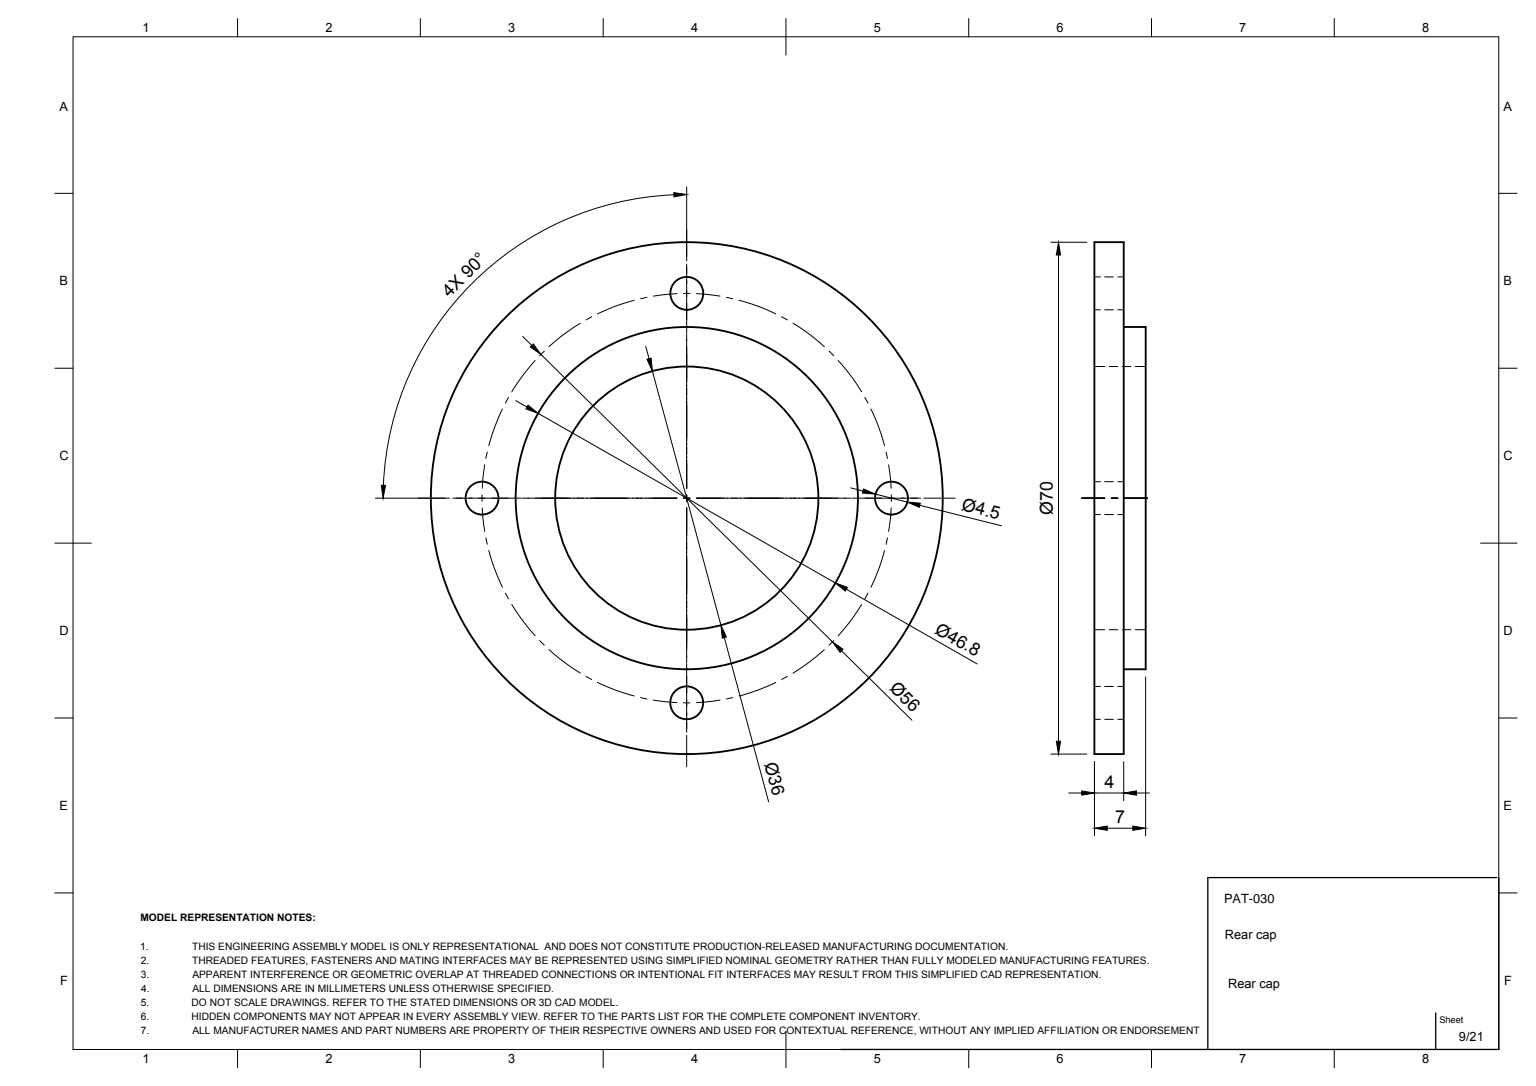
ISO-10303-21;
HEADER;
/* Generated by software containing ST-Developer
 * from STEP Tools, Inc. (www.steptools.com) 
 */

FILE_DESCRIPTION(
/* description */ ('Double-bearing flanged cartridge'),
/* implementation_level */ '2;1');

FILE_NAME(
/* name */ 'Rear cap.step',
/* time_stamp */ '2026-10-28T03:26:40-07:00',
/* author */ (''),
/* organization */ (''),
/* preprocessor_version */ 'ST-DEVELOPER v20.2',
/* originating_system */ 'Autodesk Translation Framework v15.17.0.0',
/* authorisation */ '');

FILE_SCHEMA (('AUTOMOTIVE_DESIGN { 1 0 10303 214 3 1 1 }'));
ENDSEC;

DATA;
#10=MECHANICAL_DESIGN_GEOMETRIC_PRESENTATION_REPRESENTATION('',(#207),#5535);
#171=SHAPE_REPRESENTATION_RELATIONSHIP('SRR','None',#5613,#185);
#185=ADVANCED_BREP_SHAPE_REPRESENTATION('',(#229),#5529);
#207=STYLED_ITEM('',(#5757),#229);
#229=MANIFOLD_SOLID_BREP('Body1',#2341);
#278=FACE_BOUND('',#660,.T.);
#279=FACE_BOUND('',#664,.T.);
#280=FACE_BOUND('',#665,.T.);
#281=FACE_BOUND('',#666,.T.);
#282=FACE_BOUND('',#667,.T.);
#283=FACE_BOUND('',#668,.T.);
#284=FACE_BOUND('',#670,.T.);
#285=FACE_BOUND('',#671,.T.);
#286=FACE_BOUND('',#672,.T.);
#287=FACE_BOUND('',#673,.T.);
#288=FACE_BOUND('',#674,.T.);
#337=PLANE('',#2762);
#338=PLANE('',#2769);
#339=PLANE('',#2770);
#460=FACE_OUTER_BOUND('',#654,.T.);
#461=FACE_OUTER_BOUND('',#655,.T.);
#462=FACE_OUTER_BOUND('',#656,.T.);
#463=FACE_OUTER_BOUND('',#657,.T.);
#464=FACE_OUTER_BOUND('',#658,.T.);
#465=FACE_OUTER_BOUND('',#659,.T.);
#466=FACE_OUTER_BOUND('',#661,.T.);
#467=FACE_OUTER_BOUND('',#662,.T.);
#468=FACE_OUTER_BOUND('',#663,.T.);
#469=FACE_OUTER_BOUND('',#669,.T.);
#654=EDGE_LOOP('',(#1930,#1931,#1932,#1933));
#655=EDGE_LOOP('',(#1934,#1935,#1936,#1937));
#656=EDGE_LOOP('',(#1938,#1939,#1940,#1941));
#657=EDGE_LOOP('',(#1942,#1943,#1944,#1945));
#658=EDGE_LOOP('',(#1946,#1947,#1948,#1949));
#659=EDGE_LOOP('',(#1950));
#660=EDGE_LOOP('',(#1951));
#661=EDGE_LOOP('',(#1952,#1953,#1954,#1955));
#662=EDGE_LOOP('',(#1956,#1957,#1958,#1959));
#663=EDGE_LOOP('',(#1960));
#664=EDGE_LOOP('',(#1961));
#665=EDGE_LOOP('',(#1962));
#666=EDGE_LOOP('',(#1963));
#667=EDGE_LOOP('',(#1964));
#668=EDGE_LOOP('',(#1965));
#669=EDGE_LOOP('',(#1966));
#670=EDGE_LOOP('',(#1967));
#671=EDGE_LOOP('',(#1968));
#672=EDGE_LOOP('',(#1969));
#673=EDGE_LOOP('',(#1970));
#674=EDGE_LOOP('',(#1971));
#770=LINE('',#4468,#856);
#771=LINE('',#4474,#857);
#772=LINE('',#4480,#858);
#773=LINE('',#4486,#859);
#774=LINE('',#4492,#860);
#775=LINE('',#4500,#861);
#776=LINE('',#4505,#862);
#856=VECTOR('',#3405,0.225);
#857=VECTOR('',#3412,0.225);
#858=VECTOR('',#3419,0.225);
#859=VECTOR('',#3426,0.225);
#860=VECTOR('',#3433,2.34);
#861=VECTOR('',#3444,1.8);
#862=VECTOR('',#3449,3.5);
#1026=CIRCLE('',#2748,0.225);
#1027=CIRCLE('',#2749,0.225);
#1028=CIRCLE('',#2751,0.225);
#1029=CIRCLE('',#2752,0.225);
#1030=CIRCLE('',#2754,0.225);
#1031=CIRCLE('',#2755,0.225);
#1032=CIRCLE('',#2757,0.225);
#1033=CIRCLE('',#2758,0.225);
#1034=CIRCLE('',#2760,2.34);
#1035=CIRCLE('',#2761,2.34);
#1036=CIRCLE('',#2763,1.8);
#1037=CIRCLE('',#2765,1.8);
#1038=CIRCLE('',#2767,3.5);
#1039=CIRCLE('',#2768,3.5);
#1208=VERTEX_POINT('',#4465);
#1209=VERTEX_POINT('',#4467);
#1210=VERTEX_POINT('',#4471);
#1211=VERTEX_POINT('',#4473);
#1212=VERTEX_POINT('',#4477);
#1213=VERTEX_POINT('',#4479);
#1214=VERTEX_POINT('',#4483);
#1215=VERTEX_POINT('',#4485);
#1216=VERTEX_POINT('',#4489);
#1217=VERTEX_POINT('',#4491);
#1218=VERTEX_POINT('',#4495);
#1219=VERTEX_POINT('',#4498);
#1220=VERTEX_POINT('',#4502);
#1221=VERTEX_POINT('',#4504);
#1458=EDGE_CURVE('',#1208,#1208,#1026,.T.);
#1459=EDGE_CURVE('',#1208,#1209,#770,.T.);
#1460=EDGE_CURVE('',#1209,#1209,#1027,.T.);
#1461=EDGE_CURVE('',#1210,#1210,#1028,.T.);
#1462=EDGE_CURVE('',#1210,#1211,#771,.T.);
#1463=EDGE_CURVE('',#1211,#1211,#1029,.T.);
#1464=EDGE_CURVE('',#1212,#1212,#1030,.T.);
#1465=EDGE_CURVE('',#1212,#1213,#772,.T.);
#1466=EDGE_CURVE('',#1213,#1213,#1031,.T.);
#1467=EDGE_CURVE('',#1214,#1214,#1032,.T.);
#1468=EDGE_CURVE('',#1214,#1215,#773,.T.);
#1469=EDGE_CURVE('',#1215,#1215,#1033,.T.);
#1470=EDGE_CURVE('',#1216,#1216,#1034,.T.);
#1471=EDGE_CURVE('',#1216,#1217,#774,.T.);
#1472=EDGE_CURVE('',#1217,#1217,#1035,.T.);
#1473=EDGE_CURVE('',#1218,#1218,#1036,.T.);
#1474=EDGE_CURVE('',#1219,#1219,#1037,.T.);
#1475=EDGE_CURVE('',#1219,#1218,#775,.T.);
#1476=EDGE_CURVE('',#1220,#1220,#1038,.T.);
#1477=EDGE_CURVE('',#1220,#1221,#776,.T.);
#1478=EDGE_CURVE('',#1221,#1221,#1039,.T.);
#1930=ORIENTED_EDGE('',*,*,#1458,.F.);
#1931=ORIENTED_EDGE('',*,*,#1459,.T.);
#1932=ORIENTED_EDGE('',*,*,#1460,.F.);
#1933=ORIENTED_EDGE('',*,*,#1459,.F.);
#1934=ORIENTED_EDGE('',*,*,#1461,.F.);
#1935=ORIENTED_EDGE('',*,*,#1462,.T.);
#1936=ORIENTED_EDGE('',*,*,#1463,.F.);
#1937=ORIENTED_EDGE('',*,*,#1462,.F.);
#1938=ORIENTED_EDGE('',*,*,#1464,.F.);
#1939=ORIENTED_EDGE('',*,*,#1465,.T.);
#1940=ORIENTED_EDGE('',*,*,#1466,.F.);
#1941=ORIENTED_EDGE('',*,*,#1465,.F.);
#1942=ORIENTED_EDGE('',*,*,#1467,.F.);
#1943=ORIENTED_EDGE('',*,*,#1468,.T.);
#1944=ORIENTED_EDGE('',*,*,#1469,.F.);
#1945=ORIENTED_EDGE('',*,*,#1468,.F.);
#1946=ORIENTED_EDGE('',*,*,#1470,.F.);
#1947=ORIENTED_EDGE('',*,*,#1471,.T.);
#1948=ORIENTED_EDGE('',*,*,#1472,.T.);
#1949=ORIENTED_EDGE('',*,*,#1471,.F.);
#1950=ORIENTED_EDGE('',*,*,#1472,.F.);
#1951=ORIENTED_EDGE('',*,*,#1473,.F.);
#1952=ORIENTED_EDGE('',*,*,#1474,.F.);
#1953=ORIENTED_EDGE('',*,*,#1475,.T.);
#1954=ORIENTED_EDGE('',*,*,#1473,.T.);
#1955=ORIENTED_EDGE('',*,*,#1475,.F.);
#1956=ORIENTED_EDGE('',*,*,#1476,.F.);
#1957=ORIENTED_EDGE('',*,*,#1477,.T.);
#1958=ORIENTED_EDGE('',*,*,#1478,.T.);
#1959=ORIENTED_EDGE('',*,*,#1477,.F.);
#1960=ORIENTED_EDGE('',*,*,#1476,.T.);
#1961=ORIENTED_EDGE('',*,*,#1474,.T.);
#1962=ORIENTED_EDGE('',*,*,#1469,.T.);
#1963=ORIENTED_EDGE('',*,*,#1466,.T.);
#1964=ORIENTED_EDGE('',*,*,#1463,.T.);
#1965=ORIENTED_EDGE('',*,*,#1460,.T.);
#1966=ORIENTED_EDGE('',*,*,#1478,.F.);
#1967=ORIENTED_EDGE('',*,*,#1470,.T.);
#1968=ORIENTED_EDGE('',*,*,#1467,.T.);
#1969=ORIENTED_EDGE('',*,*,#1464,.T.);
#1970=ORIENTED_EDGE('',*,*,#1461,.T.);
#1971=ORIENTED_EDGE('',*,*,#1458,.T.);
#2154=CYLINDRICAL_SURFACE('',#2747,0.225);
#2155=CYLINDRICAL_SURFACE('',#2750,0.225);
#2156=CYLINDRICAL_SURFACE('',#2753,0.225);
#2157=CYLINDRICAL_SURFACE('',#2756,0.225);
#2158=CYLINDRICAL_SURFACE('',#2759,2.34);
#2159=CYLINDRICAL_SURFACE('',#2764,1.8);
#2160=CYLINDRICAL_SURFACE('',#2766,3.5);
#2274=ADVANCED_FACE('',(#460),#2154,.F.);
#2275=ADVANCED_FACE('',(#461),#2155,.F.);
#2276=ADVANCED_FACE('',(#462),#2156,.F.);
#2277=ADVANCED_FACE('',(#463),#2157,.F.);
#2278=ADVANCED_FACE('',(#464),#2158,.T.);
#2279=ADVANCED_FACE('',(#465,#278),#337,.F.);
#2280=ADVANCED_FACE('',(#466),#2159,.F.);
#2281=ADVANCED_FACE('',(#467),#2160,.T.);
#2282=ADVANCED_FACE('',(#468,#279,#280,#281,#282,#283),#338,.T.);
#2283=ADVANCED_FACE('',(#469,#284,#285,#286,#287,#288),#339,.F.);
#2341=CLOSED_SHELL('',(#2274,#2275,#2276,#2277,#2278,#2279,#2280,#2281,
#2282,#2283));
#2746=AXIS2_PLACEMENT_3D('',#4463,#3399,#3400);
#2747=AXIS2_PLACEMENT_3D('',#4464,#3401,#3402);
#2748=AXIS2_PLACEMENT_3D('',#4466,#3403,#3404);
#2749=AXIS2_PLACEMENT_3D('',#4469,#3406,#3407);
#2750=AXIS2_PLACEMENT_3D('',#4470,#3408,#3409);
#2751=AXIS2_PLACEMENT_3D('',#4472,#3410,#3411);
#2752=AXIS2_PLACEMENT_3D('',#4475,#3413,#3414);
#2753=AXIS2_PLACEMENT_3D('',#4476,#3415,#3416);
#2754=AXIS2_PLACEMENT_3D('',#4478,#3417,#3418);
#2755=AXIS2_PLACEMENT_3D('',#4481,#3420,#3421);
#2756=AXIS2_PLACEMENT_3D('',#4482,#3422,#3423);
#2757=AXIS2_PLACEMENT_3D('',#4484,#3424,#3425);
#2758=AXIS2_PLACEMENT_3D('',#4487,#3427,#3428);
#2759=AXIS2_PLACEMENT_3D('',#4488,#3429,#3430);
#2760=AXIS2_PLACEMENT_3D('',#4490,#3431,#3432);
#2761=AXIS2_PLACEMENT_3D('',#4493,#3434,#3435);
#2762=AXIS2_PLACEMENT_3D('',#4494,#3436,#3437);
#2763=AXIS2_PLACEMENT_3D('',#4496,#3438,#3439);
#2764=AXIS2_PLACEMENT_3D('',#4497,#3440,#3441);
#2765=AXIS2_PLACEMENT_3D('',#4499,#3442,#3443);
#2766=AXIS2_PLACEMENT_3D('',#4501,#3445,#3446);
#2767=AXIS2_PLACEMENT_3D('',#4503,#3447,#3448);
#2768=AXIS2_PLACEMENT_3D('',#4506,#3450,#3451);
#2769=AXIS2_PLACEMENT_3D('',#4507,#3452,#3453);
#2770=AXIS2_PLACEMENT_3D('',#4508,#3454,#3455);
#3399=DIRECTION('axis',(0.,0.,1.));
#3400=DIRECTION('refdir',(1.,0.,0.));
#3401=DIRECTION('center_axis',(0.,1.,0.));
#3402=DIRECTION('ref_axis',(1.,0.,0.));
#3403=DIRECTION('center_axis',(0.,1.,0.));
#3404=DIRECTION('ref_axis',(1.,0.,0.));
#3405=DIRECTION('',(0.,1.,0.));
#3406=DIRECTION('center_axis',(0.,-1.,0.));
#3407=DIRECTION('ref_axis',(1.,0.,0.));
#3408=DIRECTION('center_axis',(0.,1.,0.));
#3409=DIRECTION('ref_axis',(1.,0.,0.));
#3410=DIRECTION('center_axis',(0.,1.,0.));
#3411=DIRECTION('ref_axis',(1.,0.,0.));
#3412=DIRECTION('',(0.,1.,0.));
#3413=DIRECTION('center_axis',(0.,-1.,0.));
#3414=DIRECTION('ref_axis',(1.,0.,0.));
#3415=DIRECTION('center_axis',(0.,1.,0.));
#3416=DIRECTION('ref_axis',(1.,0.,0.));
#3417=DIRECTION('center_axis',(0.,1.,0.));
#3418=DIRECTION('ref_axis',(1.,0.,0.));
#3419=DIRECTION('',(0.,1.,0.));
#3420=DIRECTION('center_axis',(0.,-1.,0.));
#3421=DIRECTION('ref_axis',(1.,0.,0.));
#3422=DIRECTION('center_axis',(0.,1.,0.));
#3423=DIRECTION('ref_axis',(1.,0.,0.));
#3424=DIRECTION('center_axis',(0.,1.,0.));
#3425=DIRECTION('ref_axis',(1.,0.,0.));
#3426=DIRECTION('',(0.,1.,0.));
#3427=DIRECTION('center_axis',(0.,-1.,0.));
#3428=DIRECTION('ref_axis',(1.,0.,0.));
#3429=DIRECTION('center_axis',(0.,1.,0.));
#3430=DIRECTION('ref_axis',(1.,0.,0.));
#3431=DIRECTION('center_axis',(0.,1.,0.));
#3432=DIRECTION('ref_axis',(1.,0.,0.));
#3433=DIRECTION('',(0.,-1.,0.));
#3434=DIRECTION('center_axis',(0.,1.,0.));
#3435=DIRECTION('ref_axis',(1.,0.,0.));
#3436=DIRECTION('center_axis',(0.,1.,0.));
#3437=DIRECTION('ref_axis',(1.,0.,0.));
#3438=DIRECTION('center_axis',(0.,-1.,0.));
#3439=DIRECTION('ref_axis',(1.,0.,0.));
#3440=DIRECTION('center_axis',(0.,1.,0.));
#3441=DIRECTION('ref_axis',(1.,0.,0.));
#3442=DIRECTION('center_axis',(0.,-1.,0.));
#3443=DIRECTION('ref_axis',(1.,0.,0.));
#3444=DIRECTION('',(0.,-1.,0.));
#3445=DIRECTION('center_axis',(0.,1.,0.));
#3446=DIRECTION('ref_axis',(1.,0.,0.));
#3447=DIRECTION('center_axis',(0.,1.,0.));
#3448=DIRECTION('ref_axis',(1.,0.,0.));
#3449=DIRECTION('',(0.,-1.,0.));
#3450=DIRECTION('center_axis',(0.,1.,0.));
#3451=DIRECTION('ref_axis',(1.,0.,0.));
#3452=DIRECTION('center_axis',(0.,1.,0.));
#3453=DIRECTION('ref_axis',(1.,0.,0.));
#3454=DIRECTION('center_axis',(0.,1.,0.));
#3455=DIRECTION('ref_axis',(1.,0.,0.));
#4463=CARTESIAN_POINT('',(0.,0.,0.));
#4464=CARTESIAN_POINT('Origin',(-2.8,5.9,4.5));
#4465=CARTESIAN_POINT('',(-3.025,6.,4.5));
#4466=CARTESIAN_POINT('Origin',(-2.8,6.,4.5));
#4467=CARTESIAN_POINT('',(-3.025,6.4,4.5));
#4468=CARTESIAN_POINT('',(-3.025,5.9,4.5));
#4469=CARTESIAN_POINT('Origin',(-2.8,6.4,4.5));
#4470=CARTESIAN_POINT('Origin',(1.71450551880629E-16,5.9,7.3));
#4471=CARTESIAN_POINT('',(-0.225,6.,7.3));
#4472=CARTESIAN_POINT('Origin',(1.71450551880629E-16,6.,7.3));
#4473=CARTESIAN_POINT('',(-0.225,6.4,7.3));
#4474=CARTESIAN_POINT('',(-0.225,5.9,7.3));
#4475=CARTESIAN_POINT('Origin',(1.71450551880629E-16,6.4,7.3));
#4476=CARTESIAN_POINT('Origin',(2.8,5.9,4.5));
#4477=CARTESIAN_POINT('',(2.575,6.,4.5));
#4478=CARTESIAN_POINT('Origin',(2.8,6.,4.5));
#4479=CARTESIAN_POINT('',(2.575,6.4,4.5));
#4480=CARTESIAN_POINT('',(2.575,5.9,4.5));
#4481=CARTESIAN_POINT('Origin',(2.8,6.4,4.5));
#4482=CARTESIAN_POINT('Origin',(-5.14351655641888E-16,5.9,1.7));
#4483=CARTESIAN_POINT('',(-0.225000000000001,6.,1.7));
#4484=CARTESIAN_POINT('Origin',(-5.14351655641888E-16,6.,1.7));
#4485=CARTESIAN_POINT('',(-0.225000000000001,6.4,1.7));
#4486=CARTESIAN_POINT('',(-0.225000000000001,5.9,1.7));
#4487=CARTESIAN_POINT('Origin',(-5.14351655641888E-16,6.4,1.7));
#4488=CARTESIAN_POINT('Origin',(0.,5.7,4.5));
#4489=CARTESIAN_POINT('',(-2.34,6.,4.5));
#4490=CARTESIAN_POINT('Origin',(0.,6.,4.5));
#4491=CARTESIAN_POINT('',(-2.34,5.7,4.5));
#4492=CARTESIAN_POINT('',(-2.34,5.7,4.5));
#4493=CARTESIAN_POINT('Origin',(0.,5.7,4.5));
#4494=CARTESIAN_POINT('Origin',(0.,5.7,4.5));
#4495=CARTESIAN_POINT('',(-1.8,5.7,4.5));
#4496=CARTESIAN_POINT('Origin',(0.,5.7,4.5));
#4497=CARTESIAN_POINT('Origin',(0.,6.,4.5));
#4498=CARTESIAN_POINT('',(-1.8,6.4,4.5));
#4499=CARTESIAN_POINT('Origin',(0.,6.4,4.5));
#4500=CARTESIAN_POINT('',(-1.8,6.,4.5));
#4501=CARTESIAN_POINT('Origin',(0.,6.,4.5));
#4502=CARTESIAN_POINT('',(-3.5,6.4,4.5));
#4503=CARTESIAN_POINT('Origin',(0.,6.4,4.5));
#4504=CARTESIAN_POINT('',(-3.5,6.,4.5));
#4505=CARTESIAN_POINT('',(-3.5,6.,4.5));
#4506=CARTESIAN_POINT('Origin',(0.,6.,4.5));
#4507=CARTESIAN_POINT('Origin',(0.,6.4,4.5));
#4508=CARTESIAN_POINT('Origin',(0.,6.,4.5));
#5510=UNCERTAINTY_MEASURE_WITH_UNIT(LENGTH_MEASURE(0.001),#5536,
'DISTANCE_ACCURACY_VALUE',
'Maximum model space distance between geometric entities at asserted c
onnectivities');
#5516=UNCERTAINTY_MEASURE_WITH_UNIT(LENGTH_MEASURE(0.001),#5536,
'DISTANCE_ACCURACY_VALUE',
'Maximum model space distance between geometric entities at asserted c
onnectivities');
#5529=(
GEOMETRIC_REPRESENTATION_CONTEXT(3)
GLOBAL_UNCERTAINTY_ASSIGNED_CONTEXT((#5510))
GLOBAL_UNIT_ASSIGNED_CONTEXT((#5536,#5538,#5539))
REPRESENTATION_CONTEXT('','3D')
);
#5535=(
GEOMETRIC_REPRESENTATION_CONTEXT(3)
GLOBAL_UNCERTAINTY_ASSIGNED_CONTEXT((#5516))
GLOBAL_UNIT_ASSIGNED_CONTEXT((#5536,#5538,#5539))
REPRESENTATION_CONTEXT('','3D')
);
#5536=(
LENGTH_UNIT()
NAMED_UNIT(*)
SI_UNIT(.CENTI.,.METRE.)
);
#5538=(
NAMED_UNIT(*)
PLANE_ANGLE_UNIT()
SI_UNIT($,.RADIAN.)
);
#5539=(
NAMED_UNIT(*)
SI_UNIT($,.STERADIAN.)
SOLID_ANGLE_UNIT()
);
#5552=SHAPE_DEFINITION_REPRESENTATION(#5575,#5613);
#5575=PRODUCT_DEFINITION_SHAPE('',$,#5632);
#5613=SHAPE_REPRESENTATION('',(#2746),#5529);
#5619=PRODUCT_DEFINITION_CONTEXT('part definition',#5675,'design');
#5632=PRODUCT_DEFINITION('Rear cap','Rear cap',#5650,#5619);
#5650=PRODUCT_DEFINITION_FORMATION('',$,#5689);
#5675=APPLICATION_CONTEXT(
'Core Data for Automotive Mechanical Design Process');
#5676=PRODUCT_CONTEXT('part definition',#5675,'mechanical');
#5689=PRODUCT('Rear cap','Rear cap','Rear cap',(#5676));
#5751=COLOUR_RGB('Sky Blue',0.24,0.69,0.87);
#5752=FILL_AREA_STYLE_COLOUR('',#5751);
#5753=FILL_AREA_STYLE('',(#5752));
#5754=SURFACE_STYLE_FILL_AREA(#5753);
#5755=SURFACE_SIDE_STYLE('',(#5754));
#5756=SURFACE_STYLE_USAGE(.BOTH.,#5755);
#5757=PRESENTATION_STYLE_ASSIGNMENT((#5756));
ENDSEC;
END-ISO-10303-21;
